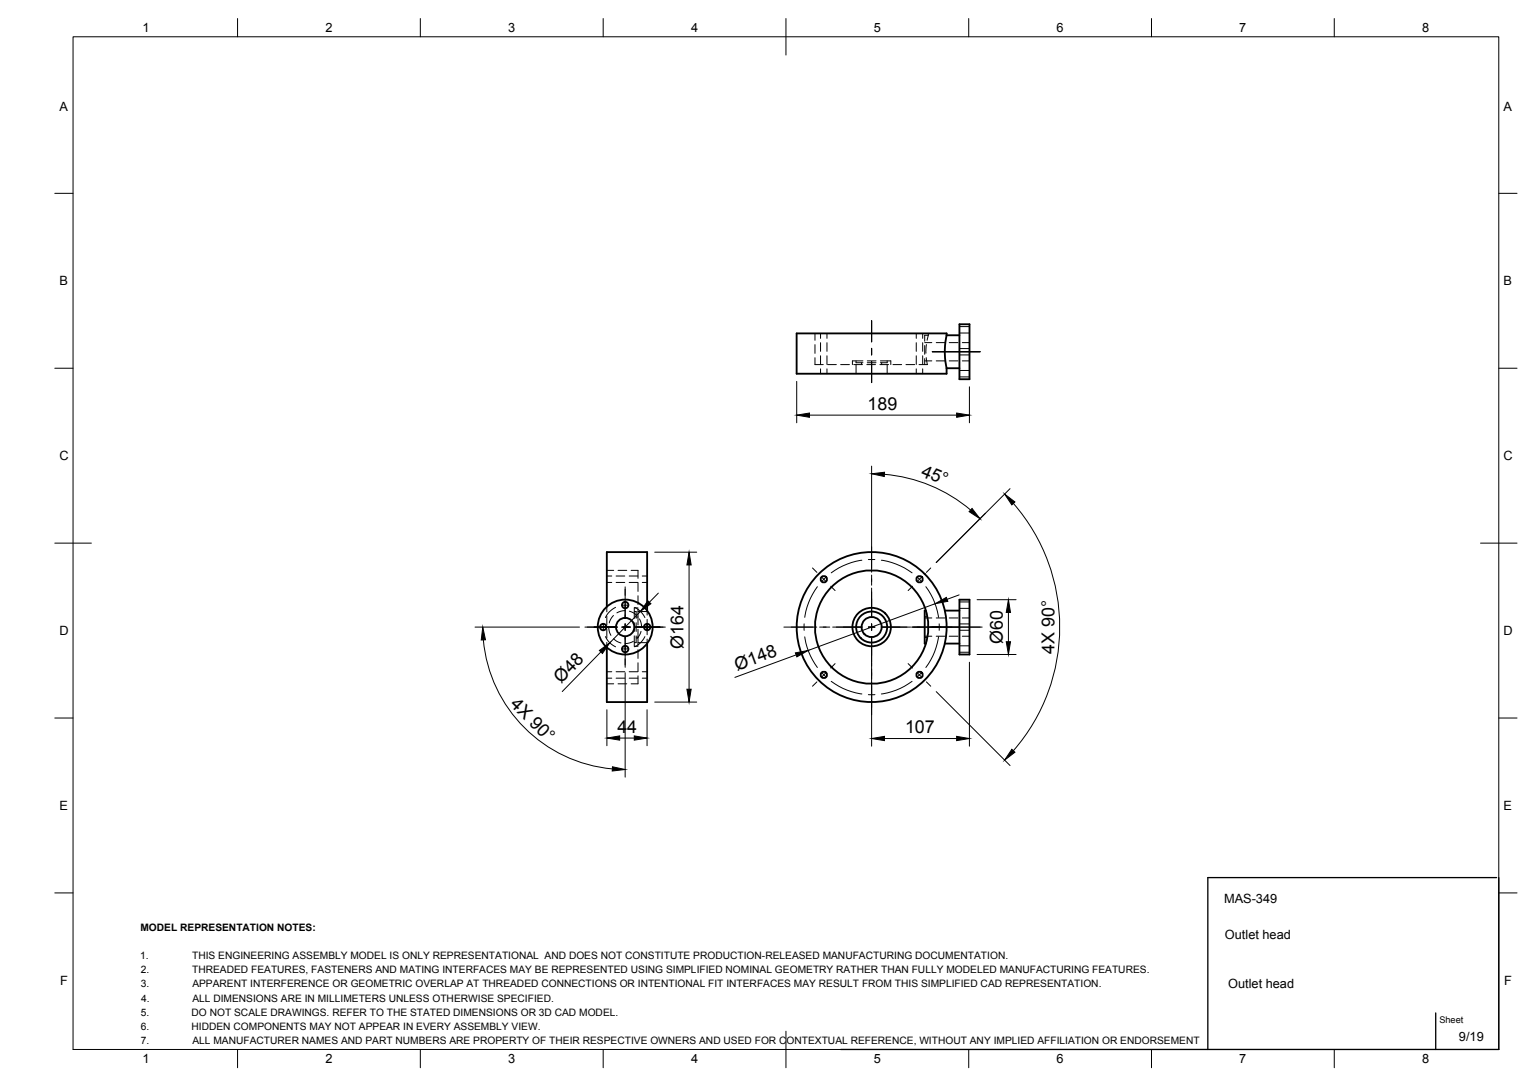
ISO-10303-21;
HEADER;
/* Generated by software containing ST-Developer
 * from STEP Tools, Inc. (www.steptools.com) 
 */

FILE_DESCRIPTION(
/* description */ ('Independent two-stage semi-open centrifugal-pump CAD. Shared impeller
s, open-machinable return casings, removable diaphragms, bronze wear/j
ournal rings, volume-preserving seal instances, retained keyed shaft, 
opposed mechanical face rings and partly threaded tie hardware. Native
 shaft rotation. Geometric topology/clearance only; flow/head/efficien
cy, pressure, cavitation, balance, preload, face loading and secondary
 seal fits/bonds, material/thermal/tolerance selection and life unassi
gned. External drive, coupling, anchors and piping bolts omitted.'),
/* implementation_level */ '2;1');

FILE_NAME(
/* name */ 'Outlet head.step',
/* time_stamp */ '2026-11-08T18:06:32-08:00',
/* author */ (''),
/* organization */ (''),
/* preprocessor_version */ 'ST-DEVELOPER v20.2',
/* originating_system */ 'Autodesk Translation Framework v15.17.0.0',
/* authorisation */ '');

FILE_SCHEMA (('AUTOMOTIVE_DESIGN { 1 0 10303 214 3 1 1 }'));
ENDSEC;

DATA;
#10=MECHANICAL_DESIGN_GEOMETRIC_PRESENTATION_REPRESENTATION('',(#399),#16687);
#308=B_SPLINE_CURVE_WITH_KNOTS('',3,(#14682,#14683,#14684,#14685,#14686,
#14687,#14688,#14689,#14690,#14691,#14692,#14693,#14694,#14695,#14696,#14697,
#14698,#14699),.UNSPECIFIED.,.F.,.F.,(4,2,2,2,2,2,2,2,4),(0.,0.340227238436096,
0.680454476872192,1.02068171530829,1.36090895374438,1.70110830750183,2.04130766125928,
2.38150701501673,2.72170636877417),.UNSPECIFIED.);
#309=B_SPLINE_CURVE_WITH_KNOTS('',3,(#14700,#14701,#14702,#14703,#14704,
#14705,#14706,#14707,#14708,#14709,#14710,#14711,#14712,#14713,#14714,#14715,
#14716,#14717,#14718,#14719,#14720,#14721,#14722,#14723,#14724,#14725,#14726,
#14727,#14728,#14729,#14730,#14731,#14732,#14733,#14734,#14735,#14736,#14737,
#14738,#14739,#14740,#14741,#14742,#14743,#14744,#14745,#14746,#14747,#14748,
#14749),.UNSPECIFIED.,.F.,.F.,(4,2,2,2,2,2,2,2,2,2,2,2,2,2,2,2,2,2,2,2,
2,2,2,2,4),(2.72170636877417,3.06190572253162,3.40210507628907,3.74230443004652,
4.08250378380397,4.42273102224006,4.76295826067616,5.10318549911225,5.44341273754835,
5.78363997598445,6.12386721442054,6.46409445285664,6.80432169129273,7.14452104505018,
7.48472039880763,7.82491975256507,8.16511910632252,8.50531846007997,8.84551781383742,
9.18571716759487,9.52591652135231,9.86614375978841,10.2063709982245,10.5465982366606,
10.8868254750967),.UNSPECIFIED.);
#310=B_SPLINE_CURVE_WITH_KNOTS('',3,(#14755,#14756,#14757,#14758,#14759,
#14760,#14761,#14762,#14763,#14764,#14765,#14766,#14767,#14768,#14769,#14770,
#14771,#14772,#14773,#14774,#14775,#14776,#14777,#14778,#14779,#14780,#14781,
#14782,#14783,#14784,#14785,#14786,#14787,#14788,#14789,#14790,#14791,#14792,
#14793,#14794,#14795,#14796,#14797,#14798,#14799,#14800,#14801,#14802,#14803,
#14804,#14805,#14806,#14807,#14808,#14809),.UNSPECIFIED.,.F.,.F.,(4,2,2,
2,2,2,2,2,2,2,2,2,2,2,2,2,2,2,2,2,2,3,2,2,2,2,4),(-7.01225091221826,-6.82312918521928,
-6.48193726869111,-6.14074535216294,-5.79955343563477,-5.4583615191066,
-5.11716960257843,-4.77597768605026,-4.43478576952209,-4.09359385299392,
-3.75249057963376,-3.41138730627361,-3.07028403291345,-2.7291807595533,
-2.38807748619315,-2.04697421283299,-1.70587093947284,-1.36476766611268,
-1.02357574958451,-0.68238383305634,-0.341191916528169,0.,0.34119191652817,
0.68238383305634,1.02357574958451,1.36476766611268,1.55388939311326),
 .UNSPECIFIED.);
#361=SHAPE_REPRESENTATION_RELATIONSHIP('SRR','None',#16770,#380);
#380=ADVANCED_BREP_SHAPE_REPRESENTATION('',(#418),#16674);
#399=STYLED_ITEM('',(#16868),#418);
#418=MANIFOLD_SOLID_BREP('Body1',#6118);
#503=FACE_BOUND('',#1324,.T.);
#504=FACE_BOUND('',#1325,.T.);
#505=FACE_BOUND('',#1326,.T.);
#506=FACE_BOUND('',#1327,.T.);
#507=FACE_BOUND('',#1328,.T.);
#508=FACE_BOUND('',#1334,.T.);
#509=FACE_BOUND('',#1335,.T.);
#510=FACE_BOUND('',#1336,.T.);
#511=FACE_BOUND('',#1337,.T.);
#512=FACE_BOUND('',#1338,.T.);
#513=FACE_BOUND('',#1341,.T.);
#514=FACE_BOUND('',#1347,.T.);
#515=FACE_BOUND('',#1354,.T.);
#516=FACE_BOUND('',#1356,.T.);
#517=FACE_BOUND('',#1360,.T.);
#518=FACE_BOUND('',#1362,.T.);
#519=FACE_BOUND('',#1365,.T.);
#520=FACE_BOUND('',#1366,.T.);
#521=FACE_BOUND('',#1367,.T.);
#522=FACE_BOUND('',#1368,.T.);
#523=FACE_BOUND('',#1369,.T.);
#524=FACE_BOUND('',#1371,.T.);
#525=FACE_BOUND('',#1372,.T.);
#526=FACE_BOUND('',#1373,.T.);
#527=FACE_BOUND('',#1374,.T.);
#528=FACE_BOUND('',#1375,.T.);
#627=PLANE('',#6716);
#628=PLANE('',#6731);
#629=PLANE('',#6735);
#630=PLANE('',#6763);
#631=PLANE('',#6765);
#632=PLANE('',#6772);
#633=PLANE('',#6773);
#634=PLANE('',#6776);
#635=PLANE('',#6777);
#904=FACE_OUTER_BOUND('',#1323,.T.);
#905=FACE_OUTER_BOUND('',#1329,.T.);
#906=FACE_OUTER_BOUND('',#1330,.T.);
#907=FACE_OUTER_BOUND('',#1331,.T.);
#908=FACE_OUTER_BOUND('',#1332,.T.);
#909=FACE_OUTER_BOUND('',#1333,.T.);
#910=FACE_OUTER_BOUND('',#1339,.T.);
#911=FACE_OUTER_BOUND('',#1340,.T.);
#912=FACE_OUTER_BOUND('',#1342,.T.);
#913=FACE_OUTER_BOUND('',#1343,.T.);
#914=FACE_OUTER_BOUND('',#1344,.T.);
#915=FACE_OUTER_BOUND('',#1345,.T.);
#916=FACE_OUTER_BOUND('',#1346,.T.);
#917=FACE_OUTER_BOUND('',#1348,.T.);
#918=FACE_OUTER_BOUND('',#1349,.T.);
#919=FACE_OUTER_BOUND('',#1350,.T.);
#920=FACE_OUTER_BOUND('',#1351,.T.);
#921=FACE_OUTER_BOUND('',#1352,.T.);
#922=FACE_OUTER_BOUND('',#1353,.T.);
#923=FACE_OUTER_BOUND('',#1355,.T.);
#924=FACE_OUTER_BOUND('',#1357,.T.);
#925=FACE_OUTER_BOUND('',#1358,.T.);
#926=FACE_OUTER_BOUND('',#1359,.T.);
#927=FACE_OUTER_BOUND('',#1361,.T.);
#928=FACE_OUTER_BOUND('',#1363,.T.);
#929=FACE_OUTER_BOUND('',#1364,.T.);
#930=FACE_OUTER_BOUND('',#1370,.T.);
#1323=EDGE_LOOP('',(#5029));
#1324=EDGE_LOOP('',(#5030));
#1325=EDGE_LOOP('',(#5031));
#1326=EDGE_LOOP('',(#5032));
#1327=EDGE_LOOP('',(#5033));
#1328=EDGE_LOOP('',(#5034));
#1329=EDGE_LOOP('',(#5035,#5036,#5037,#5038));
#1330=EDGE_LOOP('',(#5039,#5040,#5041,#5042));
#1331=EDGE_LOOP('',(#5043,#5044,#5045,#5046));
#1332=EDGE_LOOP('',(#5047,#5048,#5049,#5050));
#1333=EDGE_LOOP('',(#5051));
#1334=EDGE_LOOP('',(#5052));
#1335=EDGE_LOOP('',(#5053));
#1336=EDGE_LOOP('',(#5054));
#1337=EDGE_LOOP('',(#5055));
#1338=EDGE_LOOP('',(#5056));
#1339=EDGE_LOOP('',(#5057,#5058,#5059,#5060));
#1340=EDGE_LOOP('',(#5061,#5062));
#1341=EDGE_LOOP('',(#5063));
#1342=EDGE_LOOP('',(#5064,#5065,#5066,#5067));
#1343=EDGE_LOOP('',(#5068,#5069,#5070,#5071,#5072));
#1344=EDGE_LOOP('',(#5073,#5074,#5075,#5076));
#1345=EDGE_LOOP('',(#5077,#5078,#5079,#5080,#5081,#5082));
#1346=EDGE_LOOP('',(#5083,#5084,#5085,#5086));
#1347=EDGE_LOOP('',(#5087,#5088));
#1348=EDGE_LOOP('',(#5089,#5090,#5091,#5092));
#1349=EDGE_LOOP('',(#5093,#5094,#5095,#5096));
#1350=EDGE_LOOP('',(#5097,#5098,#5099,#5100));
#1351=EDGE_LOOP('',(#5101,#5102,#5103,#5104));
#1352=EDGE_LOOP('',(#5105,#5106,#5107,#5108));
#1353=EDGE_LOOP('',(#5109));
#1354=EDGE_LOOP('',(#5110));
#1355=EDGE_LOOP('',(#5111));
#1356=EDGE_LOOP('',(#5112));
#1357=EDGE_LOOP('',(#5113,#5114,#5115,#5116));
#1358=EDGE_LOOP('',(#5117,#5118,#5119,#5120));
#1359=EDGE_LOOP('',(#5121));
#1360=EDGE_LOOP('',(#5122));
#1361=EDGE_LOOP('',(#5123,#5124,#5125,#5126,#5127));
#1362=EDGE_LOOP('',(#5128));
#1363=EDGE_LOOP('',(#5129,#5130,#5131,#5132));
#1364=EDGE_LOOP('',(#5133));
#1365=EDGE_LOOP('',(#5134));
#1366=EDGE_LOOP('',(#5135));
#1367=EDGE_LOOP('',(#5136));
#1368=EDGE_LOOP('',(#5137));
#1369=EDGE_LOOP('',(#5138));
#1370=EDGE_LOOP('',(#5139));
#1371=EDGE_LOOP('',(#5140));
#1372=EDGE_LOOP('',(#5141));
#1373=EDGE_LOOP('',(#5142));
#1374=EDGE_LOOP('',(#5143));
#1375=EDGE_LOOP('',(#5144));
#1753=LINE('',#14648,#2122);
#1754=LINE('',#14652,#2123);
#1755=LINE('',#14656,#2124);
#1756=LINE('',#14660,#2125);
#1757=LINE('',#14668,#2126);
#1758=LINE('',#14672,#2127);
#1759=LINE('',#14677,#2128);
#1760=LINE('',#14680,#2129);
#1761=LINE('',#14752,#2130);
#1762=LINE('',#14754,#2131);
#1763=LINE('',#14814,#2132);
#1764=LINE('',#14821,#2133);
#1765=LINE('',#14827,#2134);
#1766=LINE('',#14833,#2135);
#1767=LINE('',#14839,#2136);
#1768=LINE('',#14845,#2137);
#1769=LINE('',#14851,#2138);
#1770=LINE('',#14863,#2139);
#1771=LINE('',#14868,#2140);
#1772=LINE('',#14874,#2141);
#2122=VECTOR('',#8005,0.35);
#2123=VECTOR('',#8010,0.35);
#2124=VECTOR('',#8015,0.35);
#2125=VECTOR('',#8020,0.35);
#2126=VECTOR('',#8031,3.);
#2127=VECTOR('',#8034,1.);
#2128=VECTOR('',#8041,1.);
#2129=VECTOR('',#8044,1.8);
#2130=VECTOR('',#8047,1.);
#2131=VECTOR('',#8048,1.);
#2132=VECTOR('',#8053,6.2);
#2133=VECTOR('',#8062,8.2);
#2134=VECTOR('',#8069,0.35);
#2135=VECTOR('',#8076,0.35);
#2136=VECTOR('',#8083,0.35);
#2137=VECTOR('',#8090,0.35);
#2138=VECTOR('',#8097,1.7);
#2139=VECTOR('',#8112,1.1);
#2140=VECTOR('',#8119,2.1);
#2141=VECTOR('',#8128,1.7);
#2397=CIRCLE('',#6717,3.);
#2398=CIRCLE('',#6718,0.35);
#2399=CIRCLE('',#6719,0.35);
#2400=CIRCLE('',#6720,0.35);
#2401=CIRCLE('',#6721,1.);
#2402=CIRCLE('',#6722,0.35);
#2403=CIRCLE('',#6724,0.35);
#2404=CIRCLE('',#6726,0.35);
#2405=CIRCLE('',#6728,0.35);
#2406=CIRCLE('',#6730,0.35);
#2407=CIRCLE('',#6732,3.);
#2408=CIRCLE('',#6733,1.8);
#2409=CIRCLE('',#6736,1.8);
#2410=CIRCLE('',#6737,1.);
#2411=CIRCLE('',#6742,6.2);
#2412=CIRCLE('',#6743,6.2);
#2413=CIRCLE('',#6744,6.2);
#2414=CIRCLE('',#6746,8.2);
#2415=CIRCLE('',#6747,8.2);
#2416=CIRCLE('',#6749,0.35);
#2417=CIRCLE('',#6750,0.35);
#2418=CIRCLE('',#6752,0.35);
#2419=CIRCLE('',#6753,0.35);
#2420=CIRCLE('',#6755,0.35);
#2421=CIRCLE('',#6756,0.35);
#2422=CIRCLE('',#6758,0.35);
#2423=CIRCLE('',#6759,0.35);
#2424=CIRCLE('',#6761,1.7);
#2425=CIRCLE('',#6762,1.7);
#2426=CIRCLE('',#6764,2.1);
#2427=CIRCLE('',#6766,1.7);
#2428=CIRCLE('',#6767,1.1);
#2429=CIRCLE('',#6769,1.1);
#2430=CIRCLE('',#6771,2.1);
#2431=CIRCLE('',#6775,1.7);
#2878=VERTEX_POINT('',#14634);
#2879=VERTEX_POINT('',#14636);
#2880=VERTEX_POINT('',#14638);
#2881=VERTEX_POINT('',#14640);
#2882=VERTEX_POINT('',#14642);
#2883=VERTEX_POINT('',#14644);
#2884=VERTEX_POINT('',#14647);
#2885=VERTEX_POINT('',#14651);
#2886=VERTEX_POINT('',#14655);
#2887=VERTEX_POINT('',#14659);
#2888=VERTEX_POINT('',#14663);
#2889=VERTEX_POINT('',#14665);
#2890=VERTEX_POINT('',#14670);
#2891=VERTEX_POINT('',#14671);
#2892=VERTEX_POINT('',#14674);
#2893=VERTEX_POINT('',#14679);
#2894=VERTEX_POINT('',#14681);
#2895=VERTEX_POINT('',#14751);
#2896=VERTEX_POINT('',#14753);
#2897=VERTEX_POINT('',#14811);
#2898=VERTEX_POINT('',#14813);
#2899=VERTEX_POINT('',#14818);
#2900=VERTEX_POINT('',#14820);
#2901=VERTEX_POINT('',#14824);
#2902=VERTEX_POINT('',#14826);
#2903=VERTEX_POINT('',#14830);
#2904=VERTEX_POINT('',#14832);
#2905=VERTEX_POINT('',#14836);
#2906=VERTEX_POINT('',#14838);
#2907=VERTEX_POINT('',#14842);
#2908=VERTEX_POINT('',#14844);
#2909=VERTEX_POINT('',#14848);
#2910=VERTEX_POINT('',#14850);
#2911=VERTEX_POINT('',#14854);
#2912=VERTEX_POINT('',#14857);
#2913=VERTEX_POINT('',#14859);
#2914=VERTEX_POINT('',#14862);
#2915=VERTEX_POINT('',#14866);
#2916=VERTEX_POINT('',#14872);
#3624=EDGE_CURVE('',#2878,#2878,#2397,.T.);
#3625=EDGE_CURVE('',#2879,#2879,#2398,.T.);
#3626=EDGE_CURVE('',#2880,#2880,#2399,.T.);
#3627=EDGE_CURVE('',#2881,#2881,#2400,.T.);
#3628=EDGE_CURVE('',#2882,#2882,#2401,.T.);
#3629=EDGE_CURVE('',#2883,#2883,#2402,.T.);
#3630=EDGE_CURVE('',#2881,#2884,#1753,.T.);
#3631=EDGE_CURVE('',#2884,#2884,#2403,.T.);
#3632=EDGE_CURVE('',#2883,#2885,#1754,.T.);
#3633=EDGE_CURVE('',#2885,#2885,#2404,.T.);
#3634=EDGE_CURVE('',#2879,#2886,#1755,.T.);
#3635=EDGE_CURVE('',#2886,#2886,#2405,.T.);
#3636=EDGE_CURVE('',#2880,#2887,#1756,.T.);
#3637=EDGE_CURVE('',#2887,#2887,#2406,.T.);
#3638=EDGE_CURVE('',#2888,#2888,#2407,.T.);
#3639=EDGE_CURVE('',#2889,#2889,#2408,.T.);
#3640=EDGE_CURVE('',#2878,#2888,#1757,.T.);
#3641=EDGE_CURVE('',#2890,#2891,#1758,.T.);
#3642=EDGE_CURVE('',#2891,#2890,#2409,.T.);
#3643=EDGE_CURVE('',#2892,#2892,#2410,.T.);
#3644=EDGE_CURVE('',#2882,#2892,#1759,.T.);
#3645=EDGE_CURVE('',#2889,#2893,#1760,.T.);
#3646=EDGE_CURVE('',#2894,#2893,#308,.T.);
#3647=EDGE_CURVE('',#2893,#2894,#309,.T.);
#3648=EDGE_CURVE('',#2891,#2895,#1761,.T.);
#3649=EDGE_CURVE('',#2896,#2890,#1762,.T.);
#3650=EDGE_CURVE('',#2895,#2896,#310,.T.);
#3651=EDGE_CURVE('',#2897,#2896,#2411,.T.);
#3652=EDGE_CURVE('',#2897,#2898,#1763,.T.);
#3653=EDGE_CURVE('',#2898,#2898,#2412,.T.);
#3654=EDGE_CURVE('',#2895,#2897,#2413,.T.);
#3655=EDGE_CURVE('',#2899,#2899,#2414,.T.);
#3656=EDGE_CURVE('',#2899,#2900,#1764,.T.);
#3657=EDGE_CURVE('',#2900,#2900,#2415,.T.);
#3658=EDGE_CURVE('',#2901,#2901,#2416,.T.);
#3659=EDGE_CURVE('',#2901,#2902,#1765,.T.);
#3660=EDGE_CURVE('',#2902,#2902,#2417,.T.);
#3661=EDGE_CURVE('',#2903,#2903,#2418,.T.);
#3662=EDGE_CURVE('',#2903,#2904,#1766,.T.);
#3663=EDGE_CURVE('',#2904,#2904,#2419,.T.);
#3664=EDGE_CURVE('',#2905,#2905,#2420,.T.);
#3665=EDGE_CURVE('',#2905,#2906,#1767,.T.);
#3666=EDGE_CURVE('',#2906,#2906,#2421,.T.);
#3667=EDGE_CURVE('',#2907,#2907,#2422,.T.);
#3668=EDGE_CURVE('',#2907,#2908,#1768,.T.);
#3669=EDGE_CURVE('',#2908,#2908,#2423,.T.);
#3670=EDGE_CURVE('',#2909,#2909,#2424,.T.);
#3671=EDGE_CURVE('',#2909,#2910,#1769,.T.);
#3672=EDGE_CURVE('',#2910,#2910,#2425,.T.);
#3673=EDGE_CURVE('',#2911,#2911,#2426,.T.);
#3674=EDGE_CURVE('',#2912,#2912,#2427,.T.);
#3675=EDGE_CURVE('',#2913,#2913,#2428,.T.);
#3676=EDGE_CURVE('',#2913,#2914,#1770,.T.);
#3677=EDGE_CURVE('',#2914,#2914,#2429,.T.);
#3678=EDGE_CURVE('',#2915,#2915,#2430,.T.);
#3679=EDGE_CURVE('',#2915,#2911,#1771,.T.);
#3680=EDGE_CURVE('',#2916,#2916,#2431,.T.);
#3681=EDGE_CURVE('',#2916,#2912,#1772,.T.);
#5029=ORIENTED_EDGE('',*,*,#3624,.T.);
#5030=ORIENTED_EDGE('',*,*,#3625,.T.);
#5031=ORIENTED_EDGE('',*,*,#3626,.T.);
#5032=ORIENTED_EDGE('',*,*,#3627,.T.);
#5033=ORIENTED_EDGE('',*,*,#3628,.T.);
#5034=ORIENTED_EDGE('',*,*,#3629,.T.);
#5035=ORIENTED_EDGE('',*,*,#3627,.F.);
#5036=ORIENTED_EDGE('',*,*,#3630,.T.);
#5037=ORIENTED_EDGE('',*,*,#3631,.F.);
#5038=ORIENTED_EDGE('',*,*,#3630,.F.);
#5039=ORIENTED_EDGE('',*,*,#3629,.F.);
#5040=ORIENTED_EDGE('',*,*,#3632,.T.);
#5041=ORIENTED_EDGE('',*,*,#3633,.F.);
#5042=ORIENTED_EDGE('',*,*,#3632,.F.);
#5043=ORIENTED_EDGE('',*,*,#3625,.F.);
#5044=ORIENTED_EDGE('',*,*,#3634,.T.);
#5045=ORIENTED_EDGE('',*,*,#3635,.F.);
#5046=ORIENTED_EDGE('',*,*,#3634,.F.);
#5047=ORIENTED_EDGE('',*,*,#3626,.F.);
#5048=ORIENTED_EDGE('',*,*,#3636,.T.);
#5049=ORIENTED_EDGE('',*,*,#3637,.F.);
#5050=ORIENTED_EDGE('',*,*,#3636,.F.);
#5051=ORIENTED_EDGE('',*,*,#3638,.F.);
#5052=ORIENTED_EDGE('',*,*,#3631,.T.);
#5053=ORIENTED_EDGE('',*,*,#3633,.T.);
#5054=ORIENTED_EDGE('',*,*,#3635,.T.);
#5055=ORIENTED_EDGE('',*,*,#3637,.T.);
#5056=ORIENTED_EDGE('',*,*,#3639,.T.);
#5057=ORIENTED_EDGE('',*,*,#3624,.F.);
#5058=ORIENTED_EDGE('',*,*,#3640,.T.);
#5059=ORIENTED_EDGE('',*,*,#3638,.T.);
#5060=ORIENTED_EDGE('',*,*,#3640,.F.);
#5061=ORIENTED_EDGE('',*,*,#3641,.F.);
#5062=ORIENTED_EDGE('',*,*,#3642,.F.);
#5063=ORIENTED_EDGE('',*,*,#3643,.F.);
#5064=ORIENTED_EDGE('',*,*,#3628,.F.);
#5065=ORIENTED_EDGE('',*,*,#3644,.T.);
#5066=ORIENTED_EDGE('',*,*,#3643,.T.);
#5067=ORIENTED_EDGE('',*,*,#3644,.F.);
#5068=ORIENTED_EDGE('',*,*,#3639,.F.);
#5069=ORIENTED_EDGE('',*,*,#3645,.T.);
#5070=ORIENTED_EDGE('',*,*,#3646,.F.);
#5071=ORIENTED_EDGE('',*,*,#3647,.F.);
#5072=ORIENTED_EDGE('',*,*,#3645,.F.);
#5073=ORIENTED_EDGE('',*,*,#3648,.F.);
#5074=ORIENTED_EDGE('',*,*,#3642,.T.);
#5075=ORIENTED_EDGE('',*,*,#3649,.F.);
#5076=ORIENTED_EDGE('',*,*,#3650,.F.);
#5077=ORIENTED_EDGE('',*,*,#3650,.T.);
#5078=ORIENTED_EDGE('',*,*,#3651,.F.);
#5079=ORIENTED_EDGE('',*,*,#3652,.T.);
#5080=ORIENTED_EDGE('',*,*,#3653,.T.);
#5081=ORIENTED_EDGE('',*,*,#3652,.F.);
#5082=ORIENTED_EDGE('',*,*,#3654,.F.);
#5083=ORIENTED_EDGE('',*,*,#3655,.F.);
#5084=ORIENTED_EDGE('',*,*,#3656,.T.);
#5085=ORIENTED_EDGE('',*,*,#3657,.T.);
#5086=ORIENTED_EDGE('',*,*,#3656,.F.);
#5087=ORIENTED_EDGE('',*,*,#3646,.T.);
#5088=ORIENTED_EDGE('',*,*,#3647,.T.);
#5089=ORIENTED_EDGE('',*,*,#3658,.F.);
#5090=ORIENTED_EDGE('',*,*,#3659,.T.);
#5091=ORIENTED_EDGE('',*,*,#3660,.F.);
#5092=ORIENTED_EDGE('',*,*,#3659,.F.);
#5093=ORIENTED_EDGE('',*,*,#3661,.F.);
#5094=ORIENTED_EDGE('',*,*,#3662,.T.);
#5095=ORIENTED_EDGE('',*,*,#3663,.F.);
#5096=ORIENTED_EDGE('',*,*,#3662,.F.);
#5097=ORIENTED_EDGE('',*,*,#3664,.F.);
#5098=ORIENTED_EDGE('',*,*,#3665,.T.);
#5099=ORIENTED_EDGE('',*,*,#3666,.F.);
#5100=ORIENTED_EDGE('',*,*,#3665,.F.);
#5101=ORIENTED_EDGE('',*,*,#3667,.F.);
#5102=ORIENTED_EDGE('',*,*,#3668,.T.);
#5103=ORIENTED_EDGE('',*,*,#3669,.F.);
#5104=ORIENTED_EDGE('',*,*,#3668,.F.);
#5105=ORIENTED_EDGE('',*,*,#3670,.F.);
#5106=ORIENTED_EDGE('',*,*,#3671,.T.);
#5107=ORIENTED_EDGE('',*,*,#3672,.T.);
#5108=ORIENTED_EDGE('',*,*,#3671,.F.);
#5109=ORIENTED_EDGE('',*,*,#3673,.F.);
#5110=ORIENTED_EDGE('',*,*,#3672,.F.);
#5111=ORIENTED_EDGE('',*,*,#3674,.F.);
#5112=ORIENTED_EDGE('',*,*,#3675,.T.);
#5113=ORIENTED_EDGE('',*,*,#3675,.F.);
#5114=ORIENTED_EDGE('',*,*,#3676,.T.);
#5115=ORIENTED_EDGE('',*,*,#3677,.T.);
#5116=ORIENTED_EDGE('',*,*,#3676,.F.);
#5117=ORIENTED_EDGE('',*,*,#3678,.F.);
#5118=ORIENTED_EDGE('',*,*,#3679,.T.);
#5119=ORIENTED_EDGE('',*,*,#3673,.T.);
#5120=ORIENTED_EDGE('',*,*,#3679,.F.);
#5121=ORIENTED_EDGE('',*,*,#3670,.T.);
#5122=ORIENTED_EDGE('',*,*,#3677,.F.);
#5123=ORIENTED_EDGE('',*,*,#3648,.T.);
#5124=ORIENTED_EDGE('',*,*,#3654,.T.);
#5125=ORIENTED_EDGE('',*,*,#3651,.T.);
#5126=ORIENTED_EDGE('',*,*,#3649,.T.);
#5127=ORIENTED_EDGE('',*,*,#3641,.T.);
#5128=ORIENTED_EDGE('',*,*,#3678,.T.);
#5129=ORIENTED_EDGE('',*,*,#3680,.F.);
#5130=ORIENTED_EDGE('',*,*,#3681,.T.);
#5131=ORIENTED_EDGE('',*,*,#3674,.T.);
#5132=ORIENTED_EDGE('',*,*,#3681,.F.);
#5133=ORIENTED_EDGE('',*,*,#3655,.T.);
#5134=ORIENTED_EDGE('',*,*,#3680,.T.);
#5135=ORIENTED_EDGE('',*,*,#3667,.T.);
#5136=ORIENTED_EDGE('',*,*,#3664,.T.);
#5137=ORIENTED_EDGE('',*,*,#3661,.T.);
#5138=ORIENTED_EDGE('',*,*,#3658,.T.);
#5139=ORIENTED_EDGE('',*,*,#3657,.F.);
#5140=ORIENTED_EDGE('',*,*,#3653,.F.);
#5141=ORIENTED_EDGE('',*,*,#3669,.T.);
#5142=ORIENTED_EDGE('',*,*,#3666,.T.);
#5143=ORIENTED_EDGE('',*,*,#3663,.T.);
#5144=ORIENTED_EDGE('',*,*,#3660,.T.);
#5698=CYLINDRICAL_SURFACE('',#6723,0.35);
#5699=CYLINDRICAL_SURFACE('',#6725,0.35);
#5700=CYLINDRICAL_SURFACE('',#6727,0.35);
#5701=CYLINDRICAL_SURFACE('',#6729,0.35);
#5702=CYLINDRICAL_SURFACE('',#6734,3.);
#5703=CYLINDRICAL_SURFACE('',#6738,1.);
#5704=CYLINDRICAL_SURFACE('',#6739,1.8);
#5705=CYLINDRICAL_SURFACE('',#6740,1.8);
#5706=CYLINDRICAL_SURFACE('',#6741,6.2);
#5707=CYLINDRICAL_SURFACE('',#6745,8.2);
#5708=CYLINDRICAL_SURFACE('',#6748,0.35);
#5709=CYLINDRICAL_SURFACE('',#6751,0.35);
#5710=CYLINDRICAL_SURFACE('',#6754,0.35);
#5711=CYLINDRICAL_SURFACE('',#6757,0.35);
#5712=CYLINDRICAL_SURFACE('',#6760,1.7);
#5713=CYLINDRICAL_SURFACE('',#6768,1.1);
#5714=CYLINDRICAL_SURFACE('',#6770,2.1);
#5715=CYLINDRICAL_SURFACE('',#6774,1.7);
#5983=ADVANCED_FACE('',(#904,#503,#504,#505,#506,#507),#627,.T.);
#5984=ADVANCED_FACE('',(#905),#5698,.F.);
#5985=ADVANCED_FACE('',(#906),#5699,.F.);
#5986=ADVANCED_FACE('',(#907),#5700,.F.);
#5987=ADVANCED_FACE('',(#908),#5701,.F.);
#5988=ADVANCED_FACE('',(#909,#508,#509,#510,#511,#512),#628,.F.);
#5989=ADVANCED_FACE('',(#910),#5702,.T.);
#5990=ADVANCED_FACE('',(#911,#513),#629,.F.);
#5991=ADVANCED_FACE('',(#912),#5703,.F.);
#5992=ADVANCED_FACE('',(#913),#5704,.T.);
#5993=ADVANCED_FACE('',(#914),#5705,.T.);
#5994=ADVANCED_FACE('',(#915),#5706,.F.);
#5995=ADVANCED_FACE('',(#916,#514),#5707,.T.);
#5996=ADVANCED_FACE('',(#917),#5708,.F.);
#5997=ADVANCED_FACE('',(#918),#5709,.F.);
#5998=ADVANCED_FACE('',(#919),#5710,.F.);
#5999=ADVANCED_FACE('',(#920),#5711,.F.);
#6000=ADVANCED_FACE('',(#921),#5712,.F.);
#6001=ADVANCED_FACE('',(#922,#515),#630,.F.);
#6002=ADVANCED_FACE('',(#923,#516),#631,.T.);
#6003=ADVANCED_FACE('',(#924),#5713,.F.);
#6004=ADVANCED_FACE('',(#925),#5714,.T.);
#6005=ADVANCED_FACE('',(#926,#517),#632,.F.);
#6006=ADVANCED_FACE('',(#927,#518),#633,.F.);
#6007=ADVANCED_FACE('',(#928),#5715,.F.);
#6008=ADVANCED_FACE('',(#929,#519,#520,#521,#522,#523),#634,.T.);
#6009=ADVANCED_FACE('',(#930,#524,#525,#526,#527,#528),#635,.F.);
#6118=CLOSED_SHELL('',(#5983,#5984,#5985,#5986,#5987,#5988,#5989,#5990,
#5991,#5992,#5993,#5994,#5995,#5996,#5997,#5998,#5999,#6000,#6001,#6002,
#6003,#6004,#6005,#6006,#6007,#6008,#6009));
#6715=AXIS2_PLACEMENT_3D('',#14632,#7987,#7988);
#6716=AXIS2_PLACEMENT_3D('',#14633,#7989,#7990);
#6717=AXIS2_PLACEMENT_3D('',#14635,#7991,#7992);
#6718=AXIS2_PLACEMENT_3D('',#14637,#7993,#7994);
#6719=AXIS2_PLACEMENT_3D('',#14639,#7995,#7996);
#6720=AXIS2_PLACEMENT_3D('',#14641,#7997,#7998);
#6721=AXIS2_PLACEMENT_3D('',#14643,#7999,#8000);
#6722=AXIS2_PLACEMENT_3D('',#14645,#8001,#8002);
#6723=AXIS2_PLACEMENT_3D('',#14646,#8003,#8004);
#6724=AXIS2_PLACEMENT_3D('',#14649,#8006,#8007);
#6725=AXIS2_PLACEMENT_3D('',#14650,#8008,#8009);
#6726=AXIS2_PLACEMENT_3D('',#14653,#8011,#8012);
#6727=AXIS2_PLACEMENT_3D('',#14654,#8013,#8014);
#6728=AXIS2_PLACEMENT_3D('',#14657,#8016,#8017);
#6729=AXIS2_PLACEMENT_3D('',#14658,#8018,#8019);
#6730=AXIS2_PLACEMENT_3D('',#14661,#8021,#8022);
#6731=AXIS2_PLACEMENT_3D('',#14662,#8023,#8024);
#6732=AXIS2_PLACEMENT_3D('',#14664,#8025,#8026);
#6733=AXIS2_PLACEMENT_3D('',#14666,#8027,#8028);
#6734=AXIS2_PLACEMENT_3D('',#14667,#8029,#8030);
#6735=AXIS2_PLACEMENT_3D('',#14669,#8032,#8033);
#6736=AXIS2_PLACEMENT_3D('',#14673,#8035,#8036);
#6737=AXIS2_PLACEMENT_3D('',#14675,#8037,#8038);
#6738=AXIS2_PLACEMENT_3D('',#14676,#8039,#8040);
#6739=AXIS2_PLACEMENT_3D('',#14678,#8042,#8043);
#6740=AXIS2_PLACEMENT_3D('',#14750,#8045,#8046);
#6741=AXIS2_PLACEMENT_3D('',#14810,#8049,#8050);
#6742=AXIS2_PLACEMENT_3D('',#14812,#8051,#8052);
#6743=AXIS2_PLACEMENT_3D('',#14815,#8054,#8055);
#6744=AXIS2_PLACEMENT_3D('',#14816,#8056,#8057);
#6745=AXIS2_PLACEMENT_3D('',#14817,#8058,#8059);
#6746=AXIS2_PLACEMENT_3D('',#14819,#8060,#8061);
#6747=AXIS2_PLACEMENT_3D('',#14822,#8063,#8064);
#6748=AXIS2_PLACEMENT_3D('',#14823,#8065,#8066);
#6749=AXIS2_PLACEMENT_3D('',#14825,#8067,#8068);
#6750=AXIS2_PLACEMENT_3D('',#14828,#8070,#8071);
#6751=AXIS2_PLACEMENT_3D('',#14829,#8072,#8073);
#6752=AXIS2_PLACEMENT_3D('',#14831,#8074,#8075);
#6753=AXIS2_PLACEMENT_3D('',#14834,#8077,#8078);
#6754=AXIS2_PLACEMENT_3D('',#14835,#8079,#8080);
#6755=AXIS2_PLACEMENT_3D('',#14837,#8081,#8082);
#6756=AXIS2_PLACEMENT_3D('',#14840,#8084,#8085);
#6757=AXIS2_PLACEMENT_3D('',#14841,#8086,#8087);
#6758=AXIS2_PLACEMENT_3D('',#14843,#8088,#8089);
#6759=AXIS2_PLACEMENT_3D('',#14846,#8091,#8092);
#6760=AXIS2_PLACEMENT_3D('',#14847,#8093,#8094);
#6761=AXIS2_PLACEMENT_3D('',#14849,#8095,#8096);
#6762=AXIS2_PLACEMENT_3D('',#14852,#8098,#8099);
#6763=AXIS2_PLACEMENT_3D('',#14853,#8100,#8101);
#6764=AXIS2_PLACEMENT_3D('',#14855,#8102,#8103);
#6765=AXIS2_PLACEMENT_3D('',#14856,#8104,#8105);
#6766=AXIS2_PLACEMENT_3D('',#14858,#8106,#8107);
#6767=AXIS2_PLACEMENT_3D('',#14860,#8108,#8109);
#6768=AXIS2_PLACEMENT_3D('',#14861,#8110,#8111);
#6769=AXIS2_PLACEMENT_3D('',#14864,#8113,#8114);
#6770=AXIS2_PLACEMENT_3D('',#14865,#8115,#8116);
#6771=AXIS2_PLACEMENT_3D('',#14867,#8117,#8118);
#6772=AXIS2_PLACEMENT_3D('',#14869,#8120,#8121);
#6773=AXIS2_PLACEMENT_3D('',#14870,#8122,#8123);
#6774=AXIS2_PLACEMENT_3D('',#14871,#8124,#8125);
#6775=AXIS2_PLACEMENT_3D('',#14873,#8126,#8127);
#6776=AXIS2_PLACEMENT_3D('',#14875,#8129,#8130);
#6777=AXIS2_PLACEMENT_3D('',#14876,#8131,#8132);
#7987=DIRECTION('axis',(0.,0.,1.));
#7988=DIRECTION('refdir',(1.,0.,0.));
#7989=DIRECTION('center_axis',(0.707106781186548,0.707106781186548,0.));
#7990=DIRECTION('ref_axis',(-0.707106781186548,0.707106781186548,0.));
#7991=DIRECTION('center_axis',(0.707106781186548,0.707106781186548,0.));
#7992=DIRECTION('ref_axis',(-0.707106781186547,0.707106781186547,0.));
#7993=DIRECTION('center_axis',(-0.707106781186548,-0.707106781186548,0.));
#7994=DIRECTION('ref_axis',(-0.707106781186547,0.707106781186547,0.));
#7995=DIRECTION('center_axis',(-0.707106781186548,-0.707106781186548,0.));
#7996=DIRECTION('ref_axis',(-0.707106781186547,0.707106781186547,0.));
#7997=DIRECTION('center_axis',(-0.707106781186548,-0.707106781186548,0.));
#7998=DIRECTION('ref_axis',(-0.707106781186547,0.707106781186547,0.));
#7999=DIRECTION('center_axis',(-0.707106781186548,-0.707106781186548,0.));
#8000=DIRECTION('ref_axis',(-0.707106781186548,0.707106781186548,0.));
#8001=DIRECTION('center_axis',(-0.707106781186548,-0.707106781186548,0.));
#8002=DIRECTION('ref_axis',(-0.707106781186547,0.707106781186547,0.));
#8003=DIRECTION('center_axis',(-0.707106781186548,-0.707106781186548,0.));
#8004=DIRECTION('ref_axis',(0.,0.,1.));
#8005=DIRECTION('',(-0.707106781186548,-0.707106781186548,0.));
#8006=DIRECTION('center_axis',(0.707106781186548,0.707106781186548,0.));
#8007=DIRECTION('ref_axis',(0.,0.,1.));
#8008=DIRECTION('center_axis',(-0.707106781186548,-0.707106781186548,0.));
#8009=DIRECTION('ref_axis',(0.,0.,1.));
#8010=DIRECTION('',(-0.707106781186548,-0.707106781186548,0.));
#8011=DIRECTION('center_axis',(0.707106781186548,0.707106781186548,0.));
#8012=DIRECTION('ref_axis',(0.,0.,1.));
#8013=DIRECTION('center_axis',(-0.707106781186548,-0.707106781186548,0.));
#8014=DIRECTION('ref_axis',(0.,0.,1.));
#8015=DIRECTION('',(-0.707106781186548,-0.707106781186548,0.));
#8016=DIRECTION('center_axis',(0.707106781186548,0.707106781186548,0.));
#8017=DIRECTION('ref_axis',(0.,0.,1.));
#8018=DIRECTION('center_axis',(-0.707106781186548,-0.707106781186547,3.92523114670943E-17));
#8019=DIRECTION('ref_axis',(-0.707106781186547,0.707106781186548,0.));
#8020=DIRECTION('',(-0.707106781186548,-0.707106781186547,3.92523114670943E-17));
#8021=DIRECTION('center_axis',(0.707106781186548,0.707106781186548,0.));
#8022=DIRECTION('ref_axis',(-0.707106781186547,0.707106781186548,0.));
#8023=DIRECTION('center_axis',(0.707106781186548,0.707106781186548,0.));
#8024=DIRECTION('ref_axis',(0.,0.,1.));
#8025=DIRECTION('center_axis',(0.707106781186548,0.707106781186548,0.));
#8026=DIRECTION('ref_axis',(0.,0.,1.));
#8027=DIRECTION('center_axis',(0.707106781186548,0.707106781186548,0.));
#8028=DIRECTION('ref_axis',(0.,0.,1.));
#8029=DIRECTION('center_axis',(0.707106781186548,0.707106781186548,0.));
#8030=DIRECTION('ref_axis',(0.,0.,1.));
#8031=DIRECTION('',(-0.707106781186548,-0.707106781186548,0.));
#8032=DIRECTION('center_axis',(0.707106781186548,0.707106781186548,0.));
#8033=DIRECTION('ref_axis',(0.,0.,1.));
#8034=DIRECTION('',(0.707106781186548,-0.707106781186548,0.));
#8035=DIRECTION('center_axis',(0.707106781186548,0.707106781186548,0.));
#8036=DIRECTION('ref_axis',(0.,0.,1.));
#8037=DIRECTION('center_axis',(-0.707106781186548,-0.707106781186548,0.));
#8038=DIRECTION('ref_axis',(0.,0.,1.));
#8039=DIRECTION('center_axis',(0.707106781186548,0.707106781186548,0.));
#8040=DIRECTION('ref_axis',(0.,0.,1.));
#8041=DIRECTION('',(-0.707106781186548,-0.707106781186548,0.));
#8042=DIRECTION('center_axis',(0.707106781186548,0.707106781186548,0.));
#8043=DIRECTION('ref_axis',(0.,0.,1.));
#8044=DIRECTION('',(-0.707106781186548,-0.707106781186548,0.));
#8045=DIRECTION('center_axis',(0.707106781186548,0.707106781186548,0.));
#8046=DIRECTION('ref_axis',(8.65956056235493E-17,-8.65956056235493E-17,
-1.));
#8047=DIRECTION('',(0.707106781186548,0.707106781186548,0.));
#8048=DIRECTION('',(-0.707106781186548,-0.707106781186548,0.));
#8049=DIRECTION('center_axis',(0.,0.,1.));
#8050=DIRECTION('ref_axis',(1.,0.,0.));
#8051=DIRECTION('center_axis',(0.,0.,-1.));
#8052=DIRECTION('ref_axis',(1.,0.,0.));
#8053=DIRECTION('',(0.,0.,-1.));
#8054=DIRECTION('center_axis',(0.,0.,-1.));
#8055=DIRECTION('ref_axis',(1.,0.,0.));
#8056=DIRECTION('center_axis',(0.,0.,-1.));
#8057=DIRECTION('ref_axis',(1.,0.,0.));
#8058=DIRECTION('center_axis',(0.,0.,1.));
#8059=DIRECTION('ref_axis',(1.,0.,0.));
#8060=DIRECTION('center_axis',(0.,0.,1.));
#8061=DIRECTION('ref_axis',(1.,0.,0.));
#8062=DIRECTION('',(0.,0.,-1.));
#8063=DIRECTION('center_axis',(0.,0.,1.));
#8064=DIRECTION('ref_axis',(1.,0.,0.));
#8065=DIRECTION('center_axis',(0.,0.,-1.));
#8066=DIRECTION('ref_axis',(1.,0.,0.));
#8067=DIRECTION('center_axis',(0.,0.,-1.));
#8068=DIRECTION('ref_axis',(1.,0.,0.));
#8069=DIRECTION('',(0.,0.,-1.));
#8070=DIRECTION('center_axis',(0.,0.,1.));
#8071=DIRECTION('ref_axis',(1.,0.,0.));
#8072=DIRECTION('center_axis',(0.,0.,-1.));
#8073=DIRECTION('ref_axis',(1.,0.,0.));
#8074=DIRECTION('center_axis',(0.,0.,-1.));
#8075=DIRECTION('ref_axis',(1.,0.,0.));
#8076=DIRECTION('',(0.,0.,-1.));
#8077=DIRECTION('center_axis',(0.,0.,1.));
#8078=DIRECTION('ref_axis',(1.,0.,0.));
#8079=DIRECTION('center_axis',(0.,0.,-1.));
#8080=DIRECTION('ref_axis',(1.,0.,0.));
#8081=DIRECTION('center_axis',(0.,0.,-1.));
#8082=DIRECTION('ref_axis',(1.,0.,0.));
#8083=DIRECTION('',(0.,0.,-1.));
#8084=DIRECTION('center_axis',(0.,0.,1.));
#8085=DIRECTION('ref_axis',(1.,0.,0.));
#8086=DIRECTION('center_axis',(0.,0.,-1.));
#8087=DIRECTION('ref_axis',(1.,0.,0.));
#8088=DIRECTION('center_axis',(0.,0.,-1.));
#8089=DIRECTION('ref_axis',(1.,0.,0.));
#8090=DIRECTION('',(0.,0.,-1.));
#8091=DIRECTION('center_axis',(0.,0.,1.));
#8092=DIRECTION('ref_axis',(1.,0.,0.));
#8093=DIRECTION('center_axis',(0.,0.,1.));
#8094=DIRECTION('ref_axis',(1.,0.,0.));
#8095=DIRECTION('center_axis',(0.,0.,-1.));
#8096=DIRECTION('ref_axis',(1.,0.,0.));
#8097=DIRECTION('',(0.,0.,-1.));
#8098=DIRECTION('center_axis',(0.,0.,-1.));
#8099=DIRECTION('ref_axis',(1.,0.,0.));
#8100=DIRECTION('center_axis',(0.,0.,1.));
#8101=DIRECTION('ref_axis',(1.,0.,0.));
#8102=DIRECTION('center_axis',(0.,0.,1.));
#8103=DIRECTION('ref_axis',(1.,0.,0.));
#8104=DIRECTION('center_axis',(0.,0.,1.));
#8105=DIRECTION('ref_axis',(1.,0.,0.));
#8106=DIRECTION('center_axis',(0.,0.,-1.));
#8107=DIRECTION('ref_axis',(1.,0.,0.));
#8108=DIRECTION('center_axis',(0.,0.,-1.));
#8109=DIRECTION('ref_axis',(1.,0.,0.));
#8110=DIRECTION('center_axis',(0.,0.,1.));
#8111=DIRECTION('ref_axis',(1.,0.,0.));
#8112=DIRECTION('',(0.,0.,-1.));
#8113=DIRECTION('center_axis',(0.,0.,-1.));
#8114=DIRECTION('ref_axis',(1.,0.,0.));
#8115=DIRECTION('center_axis',(0.,0.,1.));
#8116=DIRECTION('ref_axis',(1.,0.,0.));
#8117=DIRECTION('center_axis',(0.,0.,1.));
#8118=DIRECTION('ref_axis',(1.,0.,0.));
#8119=DIRECTION('',(0.,0.,-1.));
#8120=DIRECTION('center_axis',(0.,0.,1.));
#8121=DIRECTION('ref_axis',(1.,0.,0.));
#8122=DIRECTION('center_axis',(0.,0.,1.));
#8123=DIRECTION('ref_axis',(1.,0.,0.));
#8124=DIRECTION('center_axis',(0.,0.,1.));
#8125=DIRECTION('ref_axis',(1.,0.,0.));
#8126=DIRECTION('center_axis',(0.,0.,-1.));
#8127=DIRECTION('ref_axis',(1.,0.,0.));
#8128=DIRECTION('',(0.,0.,-1.));
#8129=DIRECTION('center_axis',(0.,0.,1.));
#8130=DIRECTION('ref_axis',(1.,0.,0.));
#8131=DIRECTION('center_axis',(0.,0.,1.));
#8132=DIRECTION('ref_axis',(1.,0.,0.));
#14632=CARTESIAN_POINT('',(0.,0.,0.));
#14633=CARTESIAN_POINT('Origin',(7.56604255869606,7.56604255869606,10.4));
#14634=CARTESIAN_POINT('',(7.56604255869606,7.56604255869606,7.4));
#14635=CARTESIAN_POINT('Origin',(7.56604255869606,7.56604255869606,10.4));
#14636=CARTESIAN_POINT('',(7.56604255869606,7.56604255869606,12.45));
#14637=CARTESIAN_POINT('Origin',(7.56604255869606,7.56604255869606,12.8));
#14638=CARTESIAN_POINT('',(6.11647365726364,9.01561146012848,10.4));
#14639=CARTESIAN_POINT('Origin',(5.86898628384834,9.26309883354377,10.4));
#14640=CARTESIAN_POINT('',(7.56604255869606,7.56604255869606,7.65));
#14641=CARTESIAN_POINT('Origin',(7.56604255869606,7.56604255869606,8.));
#14642=CARTESIAN_POINT('',(7.56604255869606,7.56604255869606,9.4));
#14643=CARTESIAN_POINT('Origin',(7.56604255869606,7.56604255869606,10.4));
#14644=CARTESIAN_POINT('',(9.26309883354377,5.86898628384835,10.05));
#14645=CARTESIAN_POINT('Origin',(9.26309883354377,5.86898628384834,10.4));
#14646=CARTESIAN_POINT('Origin',(7.00035713374682,7.00035713374682,8.));
#14647=CARTESIAN_POINT('',(6.78822509939086,6.78822509939086,7.65));
#14648=CARTESIAN_POINT('',(7.00035713374682,7.00035713374682,7.65));
#14649=CARTESIAN_POINT('Origin',(6.78822509939086,6.78822509939086,8.));
#14650=CARTESIAN_POINT('Origin',(8.69741340859454,5.30330085889911,10.4));
#14651=CARTESIAN_POINT('',(8.48528137423857,5.09116882454314,10.05));
#14652=CARTESIAN_POINT('',(8.69741340859454,5.30330085889911,10.05));
#14653=CARTESIAN_POINT('Origin',(8.48528137423857,5.09116882454314,10.4));
#14654=CARTESIAN_POINT('Origin',(7.00035713374682,7.00035713374682,12.8));
#14655=CARTESIAN_POINT('',(6.78822509939086,6.78822509939086,12.45));
#14656=CARTESIAN_POINT('',(7.00035713374682,7.00035713374682,12.45));
#14657=CARTESIAN_POINT('Origin',(6.78822509939086,6.78822509939086,12.8));
#14658=CARTESIAN_POINT('Origin',(5.30330085889911,8.69741340859454,10.4));
#14659=CARTESIAN_POINT('',(5.33865619795843,8.23779400082328,10.4));
#14660=CARTESIAN_POINT('',(5.5507882323144,8.44992603517924,10.4));
#14661=CARTESIAN_POINT('Origin',(5.09116882454314,8.48528137423857,10.4));
#14662=CARTESIAN_POINT('Origin',(6.78822509939086,6.78822509939086,10.4));
#14663=CARTESIAN_POINT('',(6.78822509939086,6.78822509939086,7.4));
#14664=CARTESIAN_POINT('Origin',(6.78822509939086,6.78822509939086,10.4));
#14665=CARTESIAN_POINT('',(6.78822509939086,6.78822509939086,8.6));
#14666=CARTESIAN_POINT('Origin',(6.78822509939086,6.78822509939086,10.4));
#14667=CARTESIAN_POINT('Origin',(6.78822509939086,6.78822509939086,10.4));
#14668=CARTESIAN_POINT('',(6.78822509939086,6.78822509939086,7.4));
#14669=CARTESIAN_POINT('Origin',(4.10121933088198,4.10121933088197,10.4));
#14670=CARTESIAN_POINT('',(3.30121933088198,4.90121933088198,11.8));
#14671=CARTESIAN_POINT('',(4.90121933088198,3.30121933088197,11.8));
#14672=CARTESIAN_POINT('',(4.10121933088198,4.10121933088198,11.8));
#14673=CARTESIAN_POINT('Origin',(4.10121933088198,4.10121933088197,10.4));
#14674=CARTESIAN_POINT('',(4.10121933088198,4.10121933088197,9.4));
#14675=CARTESIAN_POINT('Origin',(4.10121933088198,4.10121933088197,10.4));
#14676=CARTESIAN_POINT('Origin',(4.10121933088198,4.10121933088197,10.4));
#14677=CARTESIAN_POINT('',(4.10121933088198,4.10121933088197,9.4));
#14678=CARTESIAN_POINT('Origin',(4.10121933088198,4.10121933088197,10.4));
#14679=CARTESIAN_POINT('',(5.79827560572969,5.79827560572969,8.6));
#14680=CARTESIAN_POINT('',(4.10121933088198,4.10121933088197,8.6));
#14681=CARTESIAN_POINT('',(4.38406204335659,6.92964645562816,10.4));
#14682=CARTESIAN_POINT('Ctrl Pts',(4.38406204335659,6.92964645562816,10.4));
#14683=CARTESIAN_POINT('Ctrl Pts',(4.38406204335659,6.92964645562816,10.2865909205213));
#14684=CARTESIAN_POINT('Ctrl Pts',(4.39351442674295,6.9236969445152,10.1694312898585));
#14685=CARTESIAN_POINT('Ctrl Pts',(4.43298837551974,6.89848986805715,9.93661580499002));
#14686=CARTESIAN_POINT('Ctrl Pts',(4.46299641756371,6.87923453928561,9.82095741594961));
#14687=CARTESIAN_POINT('Ctrl Pts',(4.54148608145332,6.82767229358142,9.59933149392755));
#14688=CARTESIAN_POINT('Ctrl Pts',(4.59001683917394,6.79531113210536,9.49318037852834));
#14689=CARTESIAN_POINT('Ctrl Pts',(4.70067362633218,6.71923919982036,9.29696790693528));
#14690=CARTESIAN_POINT('Ctrl Pts',(4.762788529836,6.6755040740321,9.20690971951041));
#14691=CARTESIAN_POINT('Ctrl Pts',(4.89320891867947,6.5805026125348,9.04751240050683));
#14692=CARTESIAN_POINT('Ctrl Pts',(4.96603345147513,6.52596993125439,8.97266585747222));
#14693=CARTESIAN_POINT('Ctrl Pts',(5.12191066634055,6.40435811856043,8.84062578857748));
#14694=CARTESIAN_POINT('Ctrl Pts',(5.20494441036095,6.33726453633079,8.78342321653815));
#14695=CARTESIAN_POINT('Ctrl Pts',(5.37489594368109,6.1937760462778,8.69145891577341));
#14696=CARTESIAN_POINT('Ctrl Pts',(5.46194275097718,6.1172507384193,8.65662409391343));
#14697=CARTESIAN_POINT('Ctrl Pts',(5.63354106814756,5.95959648341559,8.61088911405032));
#14698=CARTESIAN_POINT('Ctrl Pts',(5.71808984906397,5.87846136239541,8.6));
#14699=CARTESIAN_POINT('Ctrl Pts',(5.79827560572969,5.79827560572969,8.6));
#14700=CARTESIAN_POINT('Ctrl Pts',(5.79827560572969,5.79827560572969,8.6));
#14701=CARTESIAN_POINT('Ctrl Pts',(5.87846136239541,5.71808984906396,8.6));
#14702=CARTESIAN_POINT('Ctrl Pts',(5.95959648341559,5.63354106814755,8.61088911405032));
#14703=CARTESIAN_POINT('Ctrl Pts',(6.11725073841931,5.46194275097717,8.65662409391343));
#14704=CARTESIAN_POINT('Ctrl Pts',(6.1937760462778,5.37489594368109,8.69145891577341));
#14705=CARTESIAN_POINT('Ctrl Pts',(6.3372645363308,5.20494441036095,8.78342321653815));
#14706=CARTESIAN_POINT('Ctrl Pts',(6.40435811856043,5.12191066634055,8.84062578857748));
#14707=CARTESIAN_POINT('Ctrl Pts',(6.5259699312544,4.96603345147512,8.97266585747222));
#14708=CARTESIAN_POINT('Ctrl Pts',(6.5805026125348,4.89320891867947,9.04751240050683));
#14709=CARTESIAN_POINT('Ctrl Pts',(6.6755040740321,4.76278852983599,9.20690971951041));
#14710=CARTESIAN_POINT('Ctrl Pts',(6.71923919982036,4.70067362633218,9.29696790693528));
#14711=CARTESIAN_POINT('Ctrl Pts',(6.79531113210536,4.59001683917394,9.49318037852834));
#14712=CARTESIAN_POINT('Ctrl Pts',(6.82767229358142,4.54148608145332,9.59933149392755));
#14713=CARTESIAN_POINT('Ctrl Pts',(6.87923453928561,4.46299641756371,9.82095741594961));
#14714=CARTESIAN_POINT('Ctrl Pts',(6.89848986805715,4.43298837551974,9.93661580499002));
#14715=CARTESIAN_POINT('Ctrl Pts',(6.9236969445152,4.39351442674295,10.1694312898585));
#14716=CARTESIAN_POINT('Ctrl Pts',(6.92964645562817,4.38406204335659,10.2865909205213));
#14717=CARTESIAN_POINT('Ctrl Pts',(6.92964645562817,4.38406204335659,10.5134090794787));
#14718=CARTESIAN_POINT('Ctrl Pts',(6.9236969445152,4.39351442674295,10.6305687101415));
#14719=CARTESIAN_POINT('Ctrl Pts',(6.89848986805715,4.43298837551974,10.86338419501));
#14720=CARTESIAN_POINT('Ctrl Pts',(6.87923453928561,4.46299641756371,10.9790425840504));
#14721=CARTESIAN_POINT('Ctrl Pts',(6.82767229358142,4.54148608145332,11.2006685060725));
#14722=CARTESIAN_POINT('Ctrl Pts',(6.79531113210536,4.59001683917394,11.3068196214717));
#14723=CARTESIAN_POINT('Ctrl Pts',(6.71923919982036,4.70067362633218,11.5030320930647));
#14724=CARTESIAN_POINT('Ctrl Pts',(6.6755040740321,4.76278852983599,11.5930902804896));
#14725=CARTESIAN_POINT('Ctrl Pts',(6.5805026125348,4.89320891867947,11.7524875994932));
#14726=CARTESIAN_POINT('Ctrl Pts',(6.5259699312544,4.96603345147512,11.8273341425278));
#14727=CARTESIAN_POINT('Ctrl Pts',(6.40435811856043,5.12191066634055,11.9593742114225));
#14728=CARTESIAN_POINT('Ctrl Pts',(6.3372645363308,5.20494441036095,12.0165767834619));
#14729=CARTESIAN_POINT('Ctrl Pts',(6.1937760462778,5.37489594368109,12.1085410842266));
#14730=CARTESIAN_POINT('Ctrl Pts',(6.11725073841931,5.46194275097717,12.1433759060866));
#14731=CARTESIAN_POINT('Ctrl Pts',(5.95959648341559,5.63354106814755,12.1891108859497));
#14732=CARTESIAN_POINT('Ctrl Pts',(5.87846136239541,5.71808984906396,12.2));
#14733=CARTESIAN_POINT('Ctrl Pts',(5.71808984906397,5.87846136239541,12.2));
#14734=CARTESIAN_POINT('Ctrl Pts',(5.63354106814756,5.95959648341559,12.1891108859497));
#14735=CARTESIAN_POINT('Ctrl Pts',(5.46194275097718,6.1172507384193,12.1433759060866));
#14736=CARTESIAN_POINT('Ctrl Pts',(5.37489594368109,6.19377604627779,12.1085410842266));
#14737=CARTESIAN_POINT('Ctrl Pts',(5.20494441036096,6.33726453633079,12.0165767834619));
#14738=CARTESIAN_POINT('Ctrl Pts',(5.12191066634055,6.40435811856043,11.9593742114225));
#14739=CARTESIAN_POINT('Ctrl Pts',(4.96603345147513,6.52596993125439,11.8273341425278));
#14740=CARTESIAN_POINT('Ctrl Pts',(4.89320891867947,6.5805026125348,11.7524875994932));
#14741=CARTESIAN_POINT('Ctrl Pts',(4.762788529836,6.6755040740321,11.5930902804896));
#14742=CARTESIAN_POINT('Ctrl Pts',(4.70067362633218,6.71923919982036,11.5030320930647));
#14743=CARTESIAN_POINT('Ctrl Pts',(4.59001683917394,6.79531113210536,11.3068196214717));
#14744=CARTESIAN_POINT('Ctrl Pts',(4.54148608145332,6.82767229358142,11.2006685060725));
#14745=CARTESIAN_POINT('Ctrl Pts',(4.46299641756371,6.87923453928561,10.9790425840504));
#14746=CARTESIAN_POINT('Ctrl Pts',(4.43298837551974,6.89848986805715,10.86338419501));
#14747=CARTESIAN_POINT('Ctrl Pts',(4.39351442674295,6.9236969445152,10.6305687101415));
#14748=CARTESIAN_POINT('Ctrl Pts',(4.38406204335659,6.92964645562816,10.5134090794787));
#14749=CARTESIAN_POINT('Ctrl Pts',(4.38406204335659,6.92964645562816,10.4));
#14750=CARTESIAN_POINT('Origin',(4.10121933088198,4.10121933088197,10.4));
#14751=CARTESIAN_POINT('',(5.11045241245046,3.51045241245046,11.8));
#14752=CARTESIAN_POINT('',(4.90121933088198,3.30121933088197,11.8));
#14753=CARTESIAN_POINT('',(3.51045241245046,5.11045241245046,11.8));
#14754=CARTESIAN_POINT('',(3.30121933088198,4.90121933088198,11.8));
#14755=CARTESIAN_POINT('Ctrl Pts',(5.11045241245046,3.51045241245046,11.8));
#14756=CARTESIAN_POINT('Ctrl Pts',(5.1392884847325,3.46847338586213,11.7595342292169));
#14757=CARTESIAN_POINT('Ctrl Pts',(5.16604843385166,3.42840683238517,11.7168862526028));
#14758=CARTESIAN_POINT('Ctrl Pts',(5.23513875566729,3.32263882324339,11.5932427410358));
#14759=CARTESIAN_POINT('Ctrl Pts',(5.27571579225433,3.25752083254924,11.5033547023141));
#14760=CARTESIAN_POINT('Ctrl Pts',(5.34585685398518,3.14108796317008,11.3074382155668));
#14761=CARTESIAN_POINT('Ctrl Pts',(5.37545194601955,3.08978936367632,11.2014112168311));
#14762=CARTESIAN_POINT('Ctrl Pts',(5.42242408885916,3.00659260724669,10.9798841112198));
#14763=CARTESIAN_POINT('Ctrl Pts',(5.4398572338365,2.97464720753252,10.8641950362263));
#14764=CARTESIAN_POINT('Ctrl Pts',(5.4626589384034,2.93256373453205,10.6311198770982));
#14765=CARTESIAN_POINT('Ctrl Pts',(5.46802759881639,2.92244318654482,10.5137306388427));
#14766=CARTESIAN_POINT('Ctrl Pts',(5.46802759881639,2.92244318654482,10.2862693611573));
#14767=CARTESIAN_POINT('Ctrl Pts',(5.4626589384034,2.93256373453205,10.1688801229018));
#14768=CARTESIAN_POINT('Ctrl Pts',(5.4398572338365,2.97464720753252,9.93580496377367));
#14769=CARTESIAN_POINT('Ctrl Pts',(5.42242408885916,3.00659260724669,9.82011588878015));
#14770=CARTESIAN_POINT('Ctrl Pts',(5.37545194601955,3.08978936367632,9.59858878316889));
#14771=CARTESIAN_POINT('Ctrl Pts',(5.34585685398518,3.14108796317009,9.49256178443324));
#14772=CARTESIAN_POINT('Ctrl Pts',(5.27571579225433,3.25752083254924,9.29664529768588));
#14773=CARTESIAN_POINT('Ctrl Pts',(5.23513875566729,3.32263882324339,9.20675725896418));
#14774=CARTESIAN_POINT('Ctrl Pts',(5.14624797411185,3.45871867855604,9.0476789960669));
#14775=CARTESIAN_POINT('Ctrl Pts',(5.09486035652437,3.53443821623447,8.97294373554617));
#14776=CARTESIAN_POINT('Ctrl Pts',(4.979089803435,3.69574353629806,8.84100693089275));
#14777=CARTESIAN_POINT('Ctrl Pts',(4.91468655172761,3.78130694811503,8.78379586536565));
#14778=CARTESIAN_POINT('Ctrl Pts',(4.77558243884065,3.95553264505421,8.6917407501633));
#14779=CARTESIAN_POINT('Ctrl Pts',(4.70074823922057,4.04432816738502,8.65682358615613));
#14780=CARTESIAN_POINT('Ctrl Pts',(4.54519137669676,4.21839539199965,8.61094721784197));
#14781=CARTESIAN_POINT('Ctrl Pts',(4.46446085591589,4.3036632307973,8.6));
#14782=CARTESIAN_POINT('Ctrl Pts',(4.3036632307973,4.46446085591589,8.6));
#14783=CARTESIAN_POINT('Ctrl Pts',(4.21839539199965,4.54519137669676,8.61094721784197));
#14784=CARTESIAN_POINT('Ctrl Pts',(4.04432816738502,4.70074823922057,8.65682358615613));
#14785=CARTESIAN_POINT('Ctrl Pts',(3.95553264505421,4.77558243884065,8.6917407501633));
#14786=CARTESIAN_POINT('Ctrl Pts',(3.78130694811503,4.91468655172761,8.78379586536565));
#14787=CARTESIAN_POINT('Ctrl Pts',(3.69574353629807,4.979089803435,8.84100693089275));
#14788=CARTESIAN_POINT('Ctrl Pts',(3.53443821623447,5.09486035652437,8.97294373554617));
#14789=CARTESIAN_POINT('Ctrl Pts',(3.45871867855604,5.14624797411185,9.0476789960669));
#14790=CARTESIAN_POINT('Ctrl Pts',(3.3226388232434,5.23513875566729,9.20675725896418));
#14791=CARTESIAN_POINT('Ctrl Pts',(3.25752083254925,5.27571579225433,9.29664529768588));
#14792=CARTESIAN_POINT('Ctrl Pts',(3.14108796317009,5.34585685398517,9.49256178443324));
#14793=CARTESIAN_POINT('Ctrl Pts',(3.08978936367632,5.37545194601955,9.59858878316889));
#14794=CARTESIAN_POINT('Ctrl Pts',(3.0065926072467,5.42242408885916,9.82011588878015));
#14795=CARTESIAN_POINT('Ctrl Pts',(2.97464720753252,5.4398572338365,9.93580496377367));
#14796=CARTESIAN_POINT('Ctrl Pts',(2.93256373453205,5.4626589384034,10.1688801229018));
#14797=CARTESIAN_POINT('Ctrl Pts',(2.92244318654482,5.46802759881639,10.2862693611573));
#14798=CARTESIAN_POINT('Ctrl Pts',(2.92244318654482,5.46802759881639,10.4));
#14799=CARTESIAN_POINT('Ctrl Pts',(2.92244318654482,5.46802759881639,10.5137306388427));
#14800=CARTESIAN_POINT('Ctrl Pts',(2.93256373453206,5.4626589384034,10.6311198770982));
#14801=CARTESIAN_POINT('Ctrl Pts',(2.97464720753252,5.4398572338365,10.8641950362263));
#14802=CARTESIAN_POINT('Ctrl Pts',(3.0065926072467,5.42242408885916,10.9798841112198));
#14803=CARTESIAN_POINT('Ctrl Pts',(3.08978936367632,5.37545194601955,11.2014112168311));
#14804=CARTESIAN_POINT('Ctrl Pts',(3.14108796317009,5.34585685398518,11.3074382155668));
#14805=CARTESIAN_POINT('Ctrl Pts',(3.25752083254925,5.27571579225433,11.5033547023141));
#14806=CARTESIAN_POINT('Ctrl Pts',(3.3226388232434,5.23513875566729,11.5932427410358));
#14807=CARTESIAN_POINT('Ctrl Pts',(3.42840683238549,5.16604843385145,11.7168862526031));
#14808=CARTESIAN_POINT('Ctrl Pts',(3.46847338586204,5.13928848473256,11.7595342292168));
#14809=CARTESIAN_POINT('Ctrl Pts',(3.51045241245046,5.11045241245046,11.8));
#14810=CARTESIAN_POINT('Origin',(0.,0.,8.4));
#14811=CARTESIAN_POINT('',(-6.2,-7.59281015471359E-16,11.8));
#14812=CARTESIAN_POINT('Origin',(0.,0.,11.8));
#14813=CARTESIAN_POINT('',(-6.2,-7.59281015471359E-16,8.4));
#14814=CARTESIAN_POINT('',(-6.2,-7.59281015471359E-16,8.4));
#14815=CARTESIAN_POINT('Origin',(0.,0.,8.4));
#14816=CARTESIAN_POINT('Origin',(0.,0.,11.8));
#14817=CARTESIAN_POINT('Origin',(0.,0.,8.4));
#14818=CARTESIAN_POINT('',(-8.2,-1.00421037530083E-15,12.8));
#14819=CARTESIAN_POINT('Origin',(0.,0.,12.8));
#14820=CARTESIAN_POINT('',(-8.2,-1.00421037530083E-15,8.4));
#14821=CARTESIAN_POINT('',(-8.2,-1.00421037530083E-15,8.4));
#14822=CARTESIAN_POINT('Origin',(0.,0.,8.4));
#14823=CARTESIAN_POINT('Origin',(-7.4,0.,10.6));
#14824=CARTESIAN_POINT('',(-7.75,4.28626379701574E-17,12.8));
#14825=CARTESIAN_POINT('Origin',(-7.4,0.,12.8));
#14826=CARTESIAN_POINT('',(-7.75,4.28626379701574E-17,8.4));
#14827=CARTESIAN_POINT('',(-7.75,4.28626379701574E-17,10.6));
#14828=CARTESIAN_POINT('Origin',(-7.4,0.,8.4));
#14829=CARTESIAN_POINT('Origin',(7.4,0.,10.6));
#14830=CARTESIAN_POINT('',(7.05,4.28626379701574E-17,12.8));
#14831=CARTESIAN_POINT('Origin',(7.4,0.,12.8));
#14832=CARTESIAN_POINT('',(7.05,4.28626379701574E-17,8.4));
#14833=CARTESIAN_POINT('',(7.05,4.28626379701574E-17,10.6));
#14834=CARTESIAN_POINT('Origin',(7.4,0.,8.4));
#14835=CARTESIAN_POINT('Origin',(0.,7.4,10.6));
#14836=CARTESIAN_POINT('',(-0.35,7.4,12.8));
#14837=CARTESIAN_POINT('Origin',(0.,7.4,12.8));
#14838=CARTESIAN_POINT('',(-0.35,7.4,8.4));
#14839=CARTESIAN_POINT('',(-0.35,7.4,10.6));
#14840=CARTESIAN_POINT('Origin',(0.,7.4,8.4));
#14841=CARTESIAN_POINT('Origin',(0.,-7.4,10.6));
#14842=CARTESIAN_POINT('',(-0.35,-7.4,12.8));
#14843=CARTESIAN_POINT('Origin',(0.,-7.4,12.8));
#14844=CARTESIAN_POINT('',(-0.35,-7.4,8.4));
#14845=CARTESIAN_POINT('',(-0.35,-7.4,10.6));
#14846=CARTESIAN_POINT('Origin',(0.,-7.4,8.4));
#14847=CARTESIAN_POINT('Origin',(0.,0.,11.4));
#14848=CARTESIAN_POINT('',(-1.7,-2.0818995585505E-16,11.6));
#14849=CARTESIAN_POINT('Origin',(0.,0.,11.6));
#14850=CARTESIAN_POINT('',(-1.7,-2.0818995585505E-16,11.4));
#14851=CARTESIAN_POINT('',(-1.7,-2.0818995585505E-16,11.4));
#14852=CARTESIAN_POINT('Origin',(0.,0.,11.4));
#14853=CARTESIAN_POINT('Origin',(0.,0.,11.4));
#14854=CARTESIAN_POINT('',(-2.1,-2.57175827820944E-16,11.4));
#14855=CARTESIAN_POINT('Origin',(0.,0.,11.4));
#14856=CARTESIAN_POINT('Origin',(0.,0.,11.8));
#14857=CARTESIAN_POINT('',(-1.7,-2.0818995585505E-16,11.8));
#14858=CARTESIAN_POINT('Origin',(0.,0.,11.8));
#14859=CARTESIAN_POINT('',(-1.1,-1.34711147906209E-16,11.8));
#14860=CARTESIAN_POINT('Origin',(0.,0.,11.8));
#14861=CARTESIAN_POINT('Origin',(0.,0.,11.6));
#14862=CARTESIAN_POINT('',(-1.1,-1.34711147906209E-16,11.6));
#14863=CARTESIAN_POINT('',(-1.1,-1.34711147906209E-16,11.6));
#14864=CARTESIAN_POINT('Origin',(0.,0.,11.6));
#14865=CARTESIAN_POINT('Origin',(0.,0.,11.6));
#14866=CARTESIAN_POINT('',(-2.1,-2.57175827820944E-16,11.8));
#14867=CARTESIAN_POINT('Origin',(0.,0.,11.8));
#14868=CARTESIAN_POINT('',(-2.1,-2.57175827820944E-16,11.6));
#14869=CARTESIAN_POINT('Origin',(0.,0.,11.6));
#14870=CARTESIAN_POINT('Origin',(0.,0.,11.8));
#14871=CARTESIAN_POINT('Origin',(0.,0.,11.8));
#14872=CARTESIAN_POINT('',(-1.7,-2.0818995585505E-16,12.8));
#14873=CARTESIAN_POINT('Origin',(0.,0.,12.8));
#14874=CARTESIAN_POINT('',(-1.7,-2.0818995585505E-16,11.8));
#14875=CARTESIAN_POINT('Origin',(0.,0.,12.8));
#14876=CARTESIAN_POINT('Origin',(0.,0.,8.4));
#16653=UNCERTAINTY_MEASURE_WITH_UNIT(LENGTH_MEASURE(0.001),#16688,
'DISTANCE_ACCURACY_VALUE',
'Maximum model space distance between geometric entities at asserted c
onnectivities');
#16666=UNCERTAINTY_MEASURE_WITH_UNIT(LENGTH_MEASURE(0.001),#16688,
'DISTANCE_ACCURACY_VALUE',
'Maximum model space distance between geometric entities at asserted c
onnectivities');
#16674=(
GEOMETRIC_REPRESENTATION_CONTEXT(3)
GLOBAL_UNCERTAINTY_ASSIGNED_CONTEXT((#16653))
GLOBAL_UNIT_ASSIGNED_CONTEXT((#16688,#16690,#16691))
REPRESENTATION_CONTEXT('','3D')
);
#16687=(
GEOMETRIC_REPRESENTATION_CONTEXT(3)
GLOBAL_UNCERTAINTY_ASSIGNED_CONTEXT((#16666))
GLOBAL_UNIT_ASSIGNED_CONTEXT((#16688,#16690,#16691))
REPRESENTATION_CONTEXT('','3D')
);
#16688=(
LENGTH_UNIT()
NAMED_UNIT(*)
SI_UNIT(.CENTI.,.METRE.)
);
#16690=(
NAMED_UNIT(*)
PLANE_ANGLE_UNIT()
SI_UNIT($,.RADIAN.)
);
#16691=(
NAMED_UNIT(*)
SI_UNIT($,.STERADIAN.)
SOLID_ANGLE_UNIT()
);
#16699=SHAPE_DEFINITION_REPRESENTATION(#16719,#16770);
#16719=PRODUCT_DEFINITION_SHAPE('',$,#16791);
#16770=SHAPE_REPRESENTATION('',(#6715),#16674);
#16783=PRODUCT_DEFINITION_CONTEXT('part definition',#16845,'design');
#16791=PRODUCT_DEFINITION('Outlet head','Outlet head',#16811,#16783);
#16811=PRODUCT_DEFINITION_FORMATION('',$,#16854);
#16845=APPLICATION_CONTEXT(
'Core Data for Automotive Mechanical Design Process');
#16846=PRODUCT_CONTEXT('part definition',#16845,'mechanical');
#16854=PRODUCT('Outlet head','Outlet head',$,(#16846));
#16868=PRESENTATION_STYLE_ASSIGNMENT((#16883));
#16883=SURFACE_STYLE_USAGE(.BOTH.,#16898);
#16898=SURFACE_SIDE_STYLE('',(#16913));
#16913=SURFACE_STYLE_FILL_AREA(#16928);
#16928=FILL_AREA_STYLE('Dark blue',(#16943));
#16943=FILL_AREA_STYLE_COLOUR('Dark blue',#16958);
#16958=COLOUR_RGB('Dark blue',0.0901960784313725,0.270588235294118,0.513725490196078);
ENDSEC;
END-ISO-10303-21;
